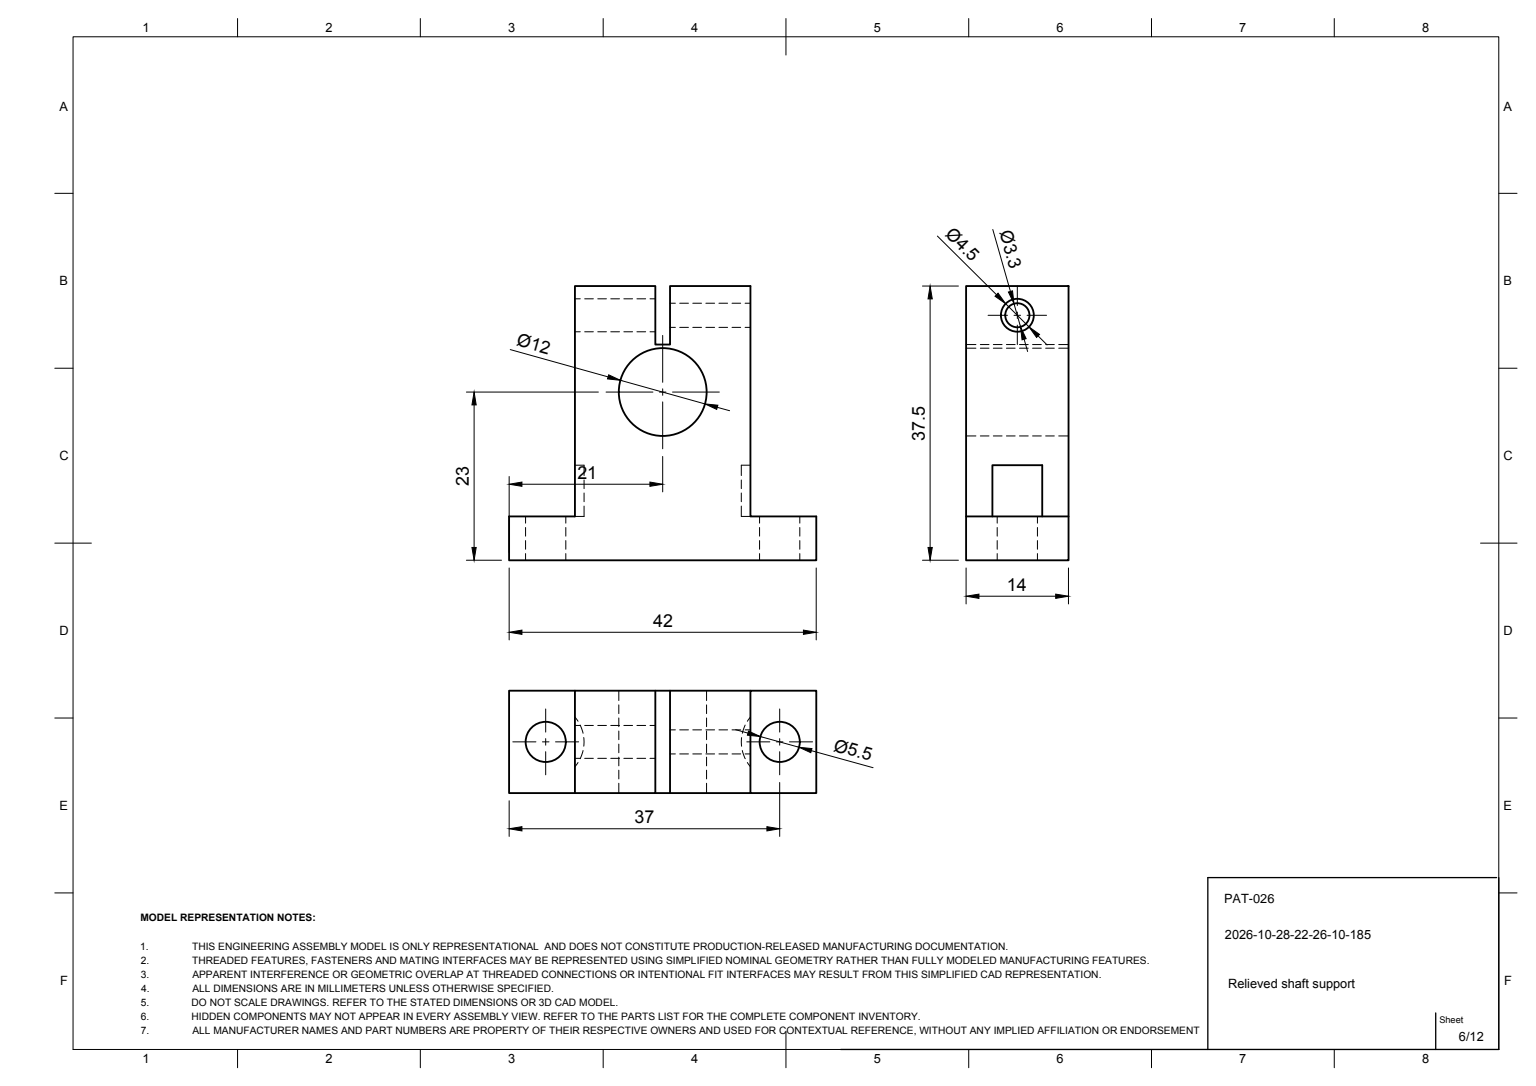
ISO-10303-21;
HEADER;
/* Generated by software containing ST-Developer
 * from STEP Tools, Inc. (www.steptools.com) 
 */

FILE_DESCRIPTION(
/* description */ ('PAT-026'),
/* implementation_level */ '2;1');

FILE_NAME(
/* name */ 'Relieved shaft support.step',
/* time_stamp */ '2026-10-28T22:25:58-07:00',
/* author */ (''),
/* organization */ (''),
/* preprocessor_version */ 'ST-DEVELOPER v20.2',
/* originating_system */ 'Autodesk Translation Framework v15.17.0.0',
/* authorisation */ '');

FILE_SCHEMA (('AUTOMOTIVE_DESIGN { 1 0 10303 214 3 1 1 }'));
ENDSEC;

DATA;
#10=MECHANICAL_DESIGN_GEOMETRIC_PRESENTATION_REPRESENTATION('',(#144),#12343);
#122=SHAPE_REPRESENTATION_RELATIONSHIP('SRR','None',#12399,#133);
#133=ADVANCED_BREP_SHAPE_REPRESENTATION('',(#155),#12334);
#144=STYLED_ITEM('',(#12533),#155);
#155=MANIFOLD_SOLID_BREP('Body1',#7350);
#169=FACE_BOUND('',#985,.T.);
#170=FACE_BOUND('',#987,.T.);
#171=FACE_BOUND('',#989,.T.);
#172=FACE_BOUND('',#996,.T.);
#173=FACE_BOUND('',#999,.T.);
#174=FACE_BOUND('',#1000,.T.);
#175=FACE_BOUND('',#1003,.T.);
#176=FACE_BOUND('',#1006,.T.);
#177=FACE_BOUND('',#1009,.T.);
#178=FACE_BOUND('',#1012,.T.);
#204=PLANE('',#7515);
#205=PLANE('',#7522);
#206=PLANE('',#7523);
#207=PLANE('',#7525);
#208=PLANE('',#7527);
#209=PLANE('',#7541);
#210=PLANE('',#7542);
#211=PLANE('',#7543);
#212=PLANE('',#7544);
#213=PLANE('',#7545);
#214=PLANE('',#7546);
#215=PLANE('',#7547);
#216=PLANE('',#7548);
#217=PLANE('',#7549);
#218=PLANE('',#7550);
#219=PLANE('',#7551);
#569=FACE_OUTER_BOUND('',#980,.T.);
#570=FACE_OUTER_BOUND('',#981,.T.);
#571=FACE_OUTER_BOUND('',#982,.T.);
#572=FACE_OUTER_BOUND('',#983,.T.);
#573=FACE_OUTER_BOUND('',#984,.T.);
#574=FACE_OUTER_BOUND('',#986,.T.);
#575=FACE_OUTER_BOUND('',#988,.T.);
#576=FACE_OUTER_BOUND('',#990,.T.);
#577=FACE_OUTER_BOUND('',#991,.T.);
#578=FACE_OUTER_BOUND('',#992,.T.);
#579=FACE_OUTER_BOUND('',#993,.T.);
#580=FACE_OUTER_BOUND('',#994,.T.);
#581=FACE_OUTER_BOUND('',#995,.T.);
#582=FACE_OUTER_BOUND('',#997,.T.);
#583=FACE_OUTER_BOUND('',#998,.T.);
#584=FACE_OUTER_BOUND('',#1001,.T.);
#585=FACE_OUTER_BOUND('',#1002,.T.);
#586=FACE_OUTER_BOUND('',#1004,.T.);
#587=FACE_OUTER_BOUND('',#1005,.T.);
#588=FACE_OUTER_BOUND('',#1007,.T.);
#589=FACE_OUTER_BOUND('',#1008,.T.);
#590=FACE_OUTER_BOUND('',#1010,.T.);
#591=FACE_OUTER_BOUND('',#1011,.T.);
#980=EDGE_LOOP('',(#4959,#4960));
#981=EDGE_LOOP('',(#4961,#4962,#4963,#4964));
#982=EDGE_LOOP('',(#4965,#4966,#4967,#4968));
#983=EDGE_LOOP('',(#4969,#4970));
#984=EDGE_LOOP('',(#4971,#4972,#4973,#4974,#4975,#4976));
#985=EDGE_LOOP('',(#4977));
#986=EDGE_LOOP('',(#4978,#4979,#4980,#4981,#4982,#4983,#4984,#4985));
#987=EDGE_LOOP('',(#4986));
#988=EDGE_LOOP('',(#4987,#4988,#4989,#4990,#4991,#4992));
#989=EDGE_LOOP('',(#4993));
#990=EDGE_LOOP('',(#4994,#4995,#4996,#4997));
#991=EDGE_LOOP('',(#4998,#4999,#5000,#5001));
#992=EDGE_LOOP('',(#5002,#5003,#5004,#5005));
#993=EDGE_LOOP('',(#5006,#5007,#5008,#5009));
#994=EDGE_LOOP('',(#5010,#5011,#5012,#5013));
#995=EDGE_LOOP('',(#5014,#5015,#5016,#5017,#5018,#5019,#5020,#5021,#5022,
#5023,#5024,#5025));
#996=EDGE_LOOP('',(#5026));
#997=EDGE_LOOP('',(#5027,#5028,#5029,#5030));
#998=EDGE_LOOP('',(#5031,#5032,#5033,#5034));
#999=EDGE_LOOP('',(#5035));
#1000=EDGE_LOOP('',(#5036));
#1001=EDGE_LOOP('',(#5037,#5038,#5039,#5040));
#1002=EDGE_LOOP('',(#5041,#5042,#5043,#5044,#5045,#5046,#5047,#5048));
#1003=EDGE_LOOP('',(#5049));
#1004=EDGE_LOOP('',(#5050,#5051,#5052,#5053));
#1005=EDGE_LOOP('',(#5054,#5055,#5056,#5057));
#1006=EDGE_LOOP('',(#5058));
#1007=EDGE_LOOP('',(#5059,#5060,#5061,#5062));
#1008=EDGE_LOOP('',(#5063,#5064,#5065,#5066));
#1009=EDGE_LOOP('',(#5067));
#1010=EDGE_LOOP('',(#5068,#5069,#5070,#5071));
#1011=EDGE_LOOP('',(#5072,#5073,#5074,#5075,#5076,#5077,#5078,#5079,#5080,
#5081,#5082,#5083));
#1012=EDGE_LOOP('',(#5084));
#1410=LINE('',#10114,#2282);
#1411=LINE('',#10118,#2283);
#1412=LINE('',#10121,#2284);
#1413=LINE('',#10125,#2285);
#1414=LINE('',#10129,#2286);
#1415=LINE('',#10132,#2287);
#1416=LINE('',#10135,#2288);
#1417=LINE('',#10137,#2289);
#1418=LINE('',#10139,#2290);
#1419=LINE('',#10141,#2291);
#1420=LINE('',#10142,#2292);
#1421=LINE('',#10147,#2293);
#1422=LINE('',#10149,#2294);
#1423=LINE('',#10150,#2295);
#1424=LINE('',#10156,#2296);
#1425=LINE('',#10158,#2297);
#1426=LINE('',#10159,#2298);
#1427=LINE('',#10161,#2299);
#1428=LINE('',#10162,#2300);
#1429=LINE('',#10169,#2301);
#1430=LINE('',#10173,#2302);
#1431=LINE('',#10178,#2303);
#1432=LINE('',#10182,#2304);
#1433=LINE('',#10187,#2305);
#1434=LINE('',#10191,#2306);
#1435=LINE('',#10193,#2307);
#1436=LINE('',#10194,#2308);
#1437=LINE('',#10196,#2309);
#1438=LINE('',#10198,#2310);
#1439=LINE('',#10200,#2311);
#1440=LINE('',#10202,#2312);
#1441=LINE('',#10204,#2313);
#1442=LINE('',#10205,#2314);
#1443=LINE('',#10208,#2315);
#1444=LINE('',#10209,#2316);
#1445=LINE('',#10212,#2317);
#1446=LINE('',#10213,#2318);
#1447=LINE('',#10215,#2319);
#1448=LINE('',#10218,#2320);
#1449=LINE('',#10219,#2321);
#1450=LINE('',#10222,#2322);
#1451=LINE('',#10223,#2323);
#1452=LINE('',#10226,#2324);
#1453=LINE('',#10227,#2325);
#1454=LINE('',#10230,#2326);
#1455=LINE('',#10231,#2327);
#1456=LINE('',#10234,#2328);
#1457=LINE('',#10235,#2329);
#1458=LINE('',#10237,#2330);
#2282=VECTOR('',#8130,1.);
#2283=VECTOR('',#8135,1.);
#2284=VECTOR('',#8138,1.);
#2285=VECTOR('',#8141,1.);
#2286=VECTOR('',#8144,1.);
#2287=VECTOR('',#8149,1.);
#2288=VECTOR('',#8152,1.);
#2289=VECTOR('',#8153,1.);
#2290=VECTOR('',#8154,1.);
#2291=VECTOR('',#8155,1.);
#2292=VECTOR('',#8156,1.);
#2293=VECTOR('',#8161,1.);
#2294=VECTOR('',#8162,1.);
#2295=VECTOR('',#8163,1.);
#2296=VECTOR('',#8168,1.);
#2297=VECTOR('',#8169,1.);
#2298=VECTOR('',#8170,1.);
#2299=VECTOR('',#8171,1.);
#2300=VECTOR('',#8172,1.);
#2301=VECTOR('',#8179,0.225);
#2302=VECTOR('',#8184,0.165);
#2303=VECTOR('',#8191,0.275);
#2304=VECTOR('',#8196,0.275);
#2305=VECTOR('',#8201,0.6);
#2306=VECTOR('',#8206,1.);
#2307=VECTOR('',#8207,1.);
#2308=VECTOR('',#8208,1.);
#2309=VECTOR('',#8209,1.);
#2310=VECTOR('',#8210,1.);
#2311=VECTOR('',#8211,1.);
#2312=VECTOR('',#8212,1.);
#2313=VECTOR('',#8213,1.);
#2314=VECTOR('',#8214,1.);
#2315=VECTOR('',#8217,1.);
#2316=VECTOR('',#8218,1.);
#2317=VECTOR('',#8221,1.);
#2318=VECTOR('',#8222,1.);
#2319=VECTOR('',#8225,1.);
#2320=VECTOR('',#8228,1.);
#2321=VECTOR('',#8229,1.);
#2322=VECTOR('',#8232,1.);
#2323=VECTOR('',#8233,1.);
#2324=VECTOR('',#8236,1.);
#2325=VECTOR('',#8237,1.);
#2326=VECTOR('',#8240,1.);
#2327=VECTOR('',#8241,1.);
#2328=VECTOR('',#8244,1.);
#2329=VECTOR('',#8245,1.);
#2330=VECTOR('',#8248,1.);
#3148=CIRCLE('',#7516,0.525);
#3149=CIRCLE('',#7518,0.525);
#3150=CIRCLE('',#7520,0.525);
#3151=CIRCLE('',#7521,0.525);
#3152=CIRCLE('',#7524,0.275);
#3153=CIRCLE('',#7526,0.165);
#3154=CIRCLE('',#7528,0.275);
#3155=CIRCLE('',#7530,0.225);
#3156=CIRCLE('',#7531,0.225);
#3157=CIRCLE('',#7533,0.165);
#3158=CIRCLE('',#7535,0.275);
#3159=CIRCLE('',#7537,0.275);
#3160=CIRCLE('',#7539,0.6);
#3161=CIRCLE('',#7540,0.6);
#3281=VERTEX_POINT('',#10112);
#3282=VERTEX_POINT('',#10113);
#3283=VERTEX_POINT('',#10117);
#3284=VERTEX_POINT('',#10119);
#3285=VERTEX_POINT('',#10123);
#3286=VERTEX_POINT('',#10124);
#3287=VERTEX_POINT('',#10126);
#3288=VERTEX_POINT('',#10128);
#3289=VERTEX_POINT('',#10134);
#3290=VERTEX_POINT('',#10136);
#3291=VERTEX_POINT('',#10138);
#3292=VERTEX_POINT('',#10140);
#3293=VERTEX_POINT('',#10143);
#3294=VERTEX_POINT('',#10146);
#3295=VERTEX_POINT('',#10148);
#3296=VERTEX_POINT('',#10151);
#3297=VERTEX_POINT('',#10154);
#3298=VERTEX_POINT('',#10155);
#3299=VERTEX_POINT('',#10157);
#3300=VERTEX_POINT('',#10160);
#3301=VERTEX_POINT('',#10163);
#3302=VERTEX_POINT('',#10166);
#3303=VERTEX_POINT('',#10168);
#3304=VERTEX_POINT('',#10172);
#3305=VERTEX_POINT('',#10176);
#3306=VERTEX_POINT('',#10180);
#3307=VERTEX_POINT('',#10184);
#3308=VERTEX_POINT('',#10186);
#3309=VERTEX_POINT('',#10190);
#3310=VERTEX_POINT('',#10192);
#3311=VERTEX_POINT('',#10195);
#3312=VERTEX_POINT('',#10197);
#3313=VERTEX_POINT('',#10199);
#3314=VERTEX_POINT('',#10201);
#3315=VERTEX_POINT('',#10203);
#3316=VERTEX_POINT('',#10207);
#3317=VERTEX_POINT('',#10211);
#3318=VERTEX_POINT('',#10217);
#3319=VERTEX_POINT('',#10221);
#3320=VERTEX_POINT('',#10225);
#3321=VERTEX_POINT('',#10229);
#3322=VERTEX_POINT('',#10233);
#3923=EDGE_CURVE('',#3281,#3282,#1410,.T.);
#3924=EDGE_CURVE('',#3282,#3281,#3148,.T.);
#3925=EDGE_CURVE('',#3283,#3281,#1411,.T.);
#3926=EDGE_CURVE('',#3284,#3283,#3149,.T.);
#3927=EDGE_CURVE('',#3282,#3284,#1412,.T.);
#3928=EDGE_CURVE('',#3285,#3286,#1413,.T.);
#3929=EDGE_CURVE('',#3285,#3287,#3150,.T.);
#3930=EDGE_CURVE('',#3288,#3287,#1414,.T.);
#3931=EDGE_CURVE('',#3286,#3288,#3151,.T.);
#3932=EDGE_CURVE('',#3287,#3285,#1415,.T.);
#3933=EDGE_CURVE('',#3283,#3289,#1416,.T.);
#3934=EDGE_CURVE('',#3290,#3289,#1417,.T.);
#3935=EDGE_CURVE('',#3290,#3291,#1418,.T.);
#3936=EDGE_CURVE('',#3292,#3291,#1419,.T.);
#3937=EDGE_CURVE('',#3292,#3284,#1420,.T.);
#3938=EDGE_CURVE('',#3293,#3293,#3152,.T.);
#3939=EDGE_CURVE('',#3294,#3292,#1421,.T.);
#3940=EDGE_CURVE('',#3294,#3295,#1422,.T.);
#3941=EDGE_CURVE('',#3289,#3295,#1423,.T.);
#3942=EDGE_CURVE('',#3296,#3296,#3153,.T.);
#3943=EDGE_CURVE('',#3297,#3298,#1424,.T.);
#3944=EDGE_CURVE('',#3299,#3298,#1425,.T.);
#3945=EDGE_CURVE('',#3286,#3299,#1426,.T.);
#3946=EDGE_CURVE('',#3300,#3288,#1427,.T.);
#3947=EDGE_CURVE('',#3297,#3300,#1428,.T.);
#3948=EDGE_CURVE('',#3301,#3301,#3154,.T.);
#3949=EDGE_CURVE('',#3302,#3302,#3155,.T.);
#3950=EDGE_CURVE('',#3302,#3303,#1429,.T.);
#3951=EDGE_CURVE('',#3303,#3303,#3156,.T.);
#3952=EDGE_CURVE('',#3296,#3304,#1430,.T.);
#3953=EDGE_CURVE('',#3304,#3304,#3157,.T.);
#3954=EDGE_CURVE('',#3305,#3305,#3158,.T.);
#3955=EDGE_CURVE('',#3305,#3293,#1431,.T.);
#3956=EDGE_CURVE('',#3306,#3306,#3159,.T.);
#3957=EDGE_CURVE('',#3306,#3301,#1432,.T.);
#3958=EDGE_CURVE('',#3307,#3307,#3160,.T.);
#3959=EDGE_CURVE('',#3307,#3308,#1433,.T.);
#3960=EDGE_CURVE('',#3308,#3308,#3161,.T.);
#3961=EDGE_CURVE('',#3291,#3309,#1434,.T.);
#3962=EDGE_CURVE('',#3309,#3310,#1435,.T.);
#3963=EDGE_CURVE('',#3310,#3297,#1436,.T.);
#3964=EDGE_CURVE('',#3300,#3311,#1437,.T.);
#3965=EDGE_CURVE('',#3311,#3312,#1438,.T.);
#3966=EDGE_CURVE('',#3312,#3313,#1439,.T.);
#3967=EDGE_CURVE('',#3313,#3314,#1440,.T.);
#3968=EDGE_CURVE('',#3314,#3315,#1441,.T.);
#3969=EDGE_CURVE('',#3315,#3294,#1442,.T.);
#3970=EDGE_CURVE('',#3316,#3290,#1443,.T.);
#3971=EDGE_CURVE('',#3309,#3316,#1444,.T.);
#3972=EDGE_CURVE('',#3317,#3316,#1445,.T.);
#3973=EDGE_CURVE('',#3310,#3317,#1446,.T.);
#3974=EDGE_CURVE('',#3298,#3317,#1447,.T.);
#3975=EDGE_CURVE('',#3318,#3299,#1448,.T.);
#3976=EDGE_CURVE('',#3311,#3318,#1449,.T.);
#3977=EDGE_CURVE('',#3319,#3318,#1450,.T.);
#3978=EDGE_CURVE('',#3312,#3319,#1451,.T.);
#3979=EDGE_CURVE('',#3320,#3319,#1452,.T.);
#3980=EDGE_CURVE('',#3313,#3320,#1453,.T.);
#3981=EDGE_CURVE('',#3321,#3320,#1454,.T.);
#3982=EDGE_CURVE('',#3314,#3321,#1455,.T.);
#3983=EDGE_CURVE('',#3322,#3321,#1456,.T.);
#3984=EDGE_CURVE('',#3315,#3322,#1457,.T.);
#3985=EDGE_CURVE('',#3295,#3322,#1458,.T.);
#4959=ORIENTED_EDGE('',*,*,#3923,.F.);
#4960=ORIENTED_EDGE('',*,*,#3924,.F.);
#4961=ORIENTED_EDGE('',*,*,#3925,.F.);
#4962=ORIENTED_EDGE('',*,*,#3926,.F.);
#4963=ORIENTED_EDGE('',*,*,#3927,.F.);
#4964=ORIENTED_EDGE('',*,*,#3924,.T.);
#4965=ORIENTED_EDGE('',*,*,#3928,.F.);
#4966=ORIENTED_EDGE('',*,*,#3929,.T.);
#4967=ORIENTED_EDGE('',*,*,#3930,.F.);
#4968=ORIENTED_EDGE('',*,*,#3931,.F.);
#4969=ORIENTED_EDGE('',*,*,#3932,.F.);
#4970=ORIENTED_EDGE('',*,*,#3929,.F.);
#4971=ORIENTED_EDGE('',*,*,#3933,.T.);
#4972=ORIENTED_EDGE('',*,*,#3934,.F.);
#4973=ORIENTED_EDGE('',*,*,#3935,.T.);
#4974=ORIENTED_EDGE('',*,*,#3936,.F.);
#4975=ORIENTED_EDGE('',*,*,#3937,.T.);
#4976=ORIENTED_EDGE('',*,*,#3926,.T.);
#4977=ORIENTED_EDGE('',*,*,#3938,.T.);
#4978=ORIENTED_EDGE('',*,*,#3925,.T.);
#4979=ORIENTED_EDGE('',*,*,#3923,.T.);
#4980=ORIENTED_EDGE('',*,*,#3927,.T.);
#4981=ORIENTED_EDGE('',*,*,#3937,.F.);
#4982=ORIENTED_EDGE('',*,*,#3939,.F.);
#4983=ORIENTED_EDGE('',*,*,#3940,.T.);
#4984=ORIENTED_EDGE('',*,*,#3941,.F.);
#4985=ORIENTED_EDGE('',*,*,#3933,.F.);
#4986=ORIENTED_EDGE('',*,*,#3942,.T.);
#4987=ORIENTED_EDGE('',*,*,#3943,.T.);
#4988=ORIENTED_EDGE('',*,*,#3944,.F.);
#4989=ORIENTED_EDGE('',*,*,#3945,.F.);
#4990=ORIENTED_EDGE('',*,*,#3931,.T.);
#4991=ORIENTED_EDGE('',*,*,#3946,.F.);
#4992=ORIENTED_EDGE('',*,*,#3947,.F.);
#4993=ORIENTED_EDGE('',*,*,#3948,.T.);
#4994=ORIENTED_EDGE('',*,*,#3949,.F.);
#4995=ORIENTED_EDGE('',*,*,#3950,.T.);
#4996=ORIENTED_EDGE('',*,*,#3951,.F.);
#4997=ORIENTED_EDGE('',*,*,#3950,.F.);
#4998=ORIENTED_EDGE('',*,*,#3942,.F.);
#4999=ORIENTED_EDGE('',*,*,#3952,.T.);
#5000=ORIENTED_EDGE('',*,*,#3953,.F.);
#5001=ORIENTED_EDGE('',*,*,#3952,.F.);
#5002=ORIENTED_EDGE('',*,*,#3954,.F.);
#5003=ORIENTED_EDGE('',*,*,#3955,.T.);
#5004=ORIENTED_EDGE('',*,*,#3938,.F.);
#5005=ORIENTED_EDGE('',*,*,#3955,.F.);
#5006=ORIENTED_EDGE('',*,*,#3956,.F.);
#5007=ORIENTED_EDGE('',*,*,#3957,.T.);
#5008=ORIENTED_EDGE('',*,*,#3948,.F.);
#5009=ORIENTED_EDGE('',*,*,#3957,.F.);
#5010=ORIENTED_EDGE('',*,*,#3958,.F.);
#5011=ORIENTED_EDGE('',*,*,#3959,.T.);
#5012=ORIENTED_EDGE('',*,*,#3960,.F.);
#5013=ORIENTED_EDGE('',*,*,#3959,.F.);
#5014=ORIENTED_EDGE('',*,*,#3936,.T.);
#5015=ORIENTED_EDGE('',*,*,#3961,.T.);
#5016=ORIENTED_EDGE('',*,*,#3962,.T.);
#5017=ORIENTED_EDGE('',*,*,#3963,.T.);
#5018=ORIENTED_EDGE('',*,*,#3947,.T.);
#5019=ORIENTED_EDGE('',*,*,#3964,.T.);
#5020=ORIENTED_EDGE('',*,*,#3965,.T.);
#5021=ORIENTED_EDGE('',*,*,#3966,.T.);
#5022=ORIENTED_EDGE('',*,*,#3967,.T.);
#5023=ORIENTED_EDGE('',*,*,#3968,.T.);
#5024=ORIENTED_EDGE('',*,*,#3969,.T.);
#5025=ORIENTED_EDGE('',*,*,#3939,.T.);
#5026=ORIENTED_EDGE('',*,*,#3958,.T.);
#5027=ORIENTED_EDGE('',*,*,#3935,.F.);
#5028=ORIENTED_EDGE('',*,*,#3970,.F.);
#5029=ORIENTED_EDGE('',*,*,#3971,.F.);
#5030=ORIENTED_EDGE('',*,*,#3961,.F.);
#5031=ORIENTED_EDGE('',*,*,#3971,.T.);
#5032=ORIENTED_EDGE('',*,*,#3972,.F.);
#5033=ORIENTED_EDGE('',*,*,#3973,.F.);
#5034=ORIENTED_EDGE('',*,*,#3962,.F.);
#5035=ORIENTED_EDGE('',*,*,#3954,.T.);
#5036=ORIENTED_EDGE('',*,*,#3956,.T.);
#5037=ORIENTED_EDGE('',*,*,#3973,.T.);
#5038=ORIENTED_EDGE('',*,*,#3974,.F.);
#5039=ORIENTED_EDGE('',*,*,#3943,.F.);
#5040=ORIENTED_EDGE('',*,*,#3963,.F.);
#5041=ORIENTED_EDGE('',*,*,#3928,.T.);
#5042=ORIENTED_EDGE('',*,*,#3945,.T.);
#5043=ORIENTED_EDGE('',*,*,#3975,.F.);
#5044=ORIENTED_EDGE('',*,*,#3976,.F.);
#5045=ORIENTED_EDGE('',*,*,#3964,.F.);
#5046=ORIENTED_EDGE('',*,*,#3946,.T.);
#5047=ORIENTED_EDGE('',*,*,#3930,.T.);
#5048=ORIENTED_EDGE('',*,*,#3932,.T.);
#5049=ORIENTED_EDGE('',*,*,#3951,.T.);
#5050=ORIENTED_EDGE('',*,*,#3976,.T.);
#5051=ORIENTED_EDGE('',*,*,#3977,.F.);
#5052=ORIENTED_EDGE('',*,*,#3978,.F.);
#5053=ORIENTED_EDGE('',*,*,#3965,.F.);
#5054=ORIENTED_EDGE('',*,*,#3978,.T.);
#5055=ORIENTED_EDGE('',*,*,#3979,.F.);
#5056=ORIENTED_EDGE('',*,*,#3980,.F.);
#5057=ORIENTED_EDGE('',*,*,#3966,.F.);
#5058=ORIENTED_EDGE('',*,*,#3949,.T.);
#5059=ORIENTED_EDGE('',*,*,#3980,.T.);
#5060=ORIENTED_EDGE('',*,*,#3981,.F.);
#5061=ORIENTED_EDGE('',*,*,#3982,.F.);
#5062=ORIENTED_EDGE('',*,*,#3967,.F.);
#5063=ORIENTED_EDGE('',*,*,#3982,.T.);
#5064=ORIENTED_EDGE('',*,*,#3983,.F.);
#5065=ORIENTED_EDGE('',*,*,#3984,.F.);
#5066=ORIENTED_EDGE('',*,*,#3968,.F.);
#5067=ORIENTED_EDGE('',*,*,#3953,.T.);
#5068=ORIENTED_EDGE('',*,*,#3984,.T.);
#5069=ORIENTED_EDGE('',*,*,#3985,.F.);
#5070=ORIENTED_EDGE('',*,*,#3940,.F.);
#5071=ORIENTED_EDGE('',*,*,#3969,.F.);
#5072=ORIENTED_EDGE('',*,*,#3934,.T.);
#5073=ORIENTED_EDGE('',*,*,#3941,.T.);
#5074=ORIENTED_EDGE('',*,*,#3985,.T.);
#5075=ORIENTED_EDGE('',*,*,#3983,.T.);
#5076=ORIENTED_EDGE('',*,*,#3981,.T.);
#5077=ORIENTED_EDGE('',*,*,#3979,.T.);
#5078=ORIENTED_EDGE('',*,*,#3977,.T.);
#5079=ORIENTED_EDGE('',*,*,#3975,.T.);
#5080=ORIENTED_EDGE('',*,*,#3944,.T.);
#5081=ORIENTED_EDGE('',*,*,#3974,.T.);
#5082=ORIENTED_EDGE('',*,*,#3972,.T.);
#5083=ORIENTED_EDGE('',*,*,#3970,.T.);
#5084=ORIENTED_EDGE('',*,*,#3960,.T.);
#6917=CYLINDRICAL_SURFACE('',#7517,0.525);
#6918=CYLINDRICAL_SURFACE('',#7519,0.525);
#6919=CYLINDRICAL_SURFACE('',#7529,0.225);
#6920=CYLINDRICAL_SURFACE('',#7532,0.165);
#6921=CYLINDRICAL_SURFACE('',#7534,0.275);
#6922=CYLINDRICAL_SURFACE('',#7536,0.275);
#6923=CYLINDRICAL_SURFACE('',#7538,0.6);
#6960=ADVANCED_FACE('',(#569),#204,.F.);
#6961=ADVANCED_FACE('',(#570),#6917,.F.);
#6962=ADVANCED_FACE('',(#571),#6918,.F.);
#6963=ADVANCED_FACE('',(#572),#205,.F.);
#6964=ADVANCED_FACE('',(#573,#169),#206,.T.);
#6965=ADVANCED_FACE('',(#574,#170),#207,.T.);
#6966=ADVANCED_FACE('',(#575,#171),#208,.T.);
#6967=ADVANCED_FACE('',(#576),#6919,.F.);
#6968=ADVANCED_FACE('',(#577),#6920,.F.);
#6969=ADVANCED_FACE('',(#578),#6921,.F.);
#6970=ADVANCED_FACE('',(#579),#6922,.F.);
#6971=ADVANCED_FACE('',(#580),#6923,.F.);
#6972=ADVANCED_FACE('',(#581,#172),#209,.T.);
#6973=ADVANCED_FACE('',(#582),#210,.T.);
#6974=ADVANCED_FACE('',(#583,#173,#174),#211,.T.);
#6975=ADVANCED_FACE('',(#584),#212,.T.);
#6976=ADVANCED_FACE('',(#585,#175),#213,.T.);
#6977=ADVANCED_FACE('',(#586),#214,.T.);
#6978=ADVANCED_FACE('',(#587,#176),#215,.T.);
#6979=ADVANCED_FACE('',(#588),#216,.T.);
#6980=ADVANCED_FACE('',(#589,#177),#217,.T.);
#6981=ADVANCED_FACE('',(#590),#218,.T.);
#6982=ADVANCED_FACE('',(#591,#178),#219,.T.);
#7350=CLOSED_SHELL('',(#6960,#6961,#6962,#6963,#6964,#6965,#6966,#6967,
#6968,#6969,#6970,#6971,#6972,#6973,#6974,#6975,#6976,#6977,#6978,#6979,
#6980,#6981,#6982));
#7514=AXIS2_PLACEMENT_3D('',#10110,#8126,#8127);
#7515=AXIS2_PLACEMENT_3D('',#10111,#8128,#8129);
#7516=AXIS2_PLACEMENT_3D('',#10115,#8131,#8132);
#7517=AXIS2_PLACEMENT_3D('',#10116,#8133,#8134);
#7518=AXIS2_PLACEMENT_3D('',#10120,#8136,#8137);
#7519=AXIS2_PLACEMENT_3D('',#10122,#8139,#8140);
#7520=AXIS2_PLACEMENT_3D('',#10127,#8142,#8143);
#7521=AXIS2_PLACEMENT_3D('',#10130,#8145,#8146);
#7522=AXIS2_PLACEMENT_3D('',#10131,#8147,#8148);
#7523=AXIS2_PLACEMENT_3D('',#10133,#8150,#8151);
#7524=AXIS2_PLACEMENT_3D('',#10144,#8157,#8158);
#7525=AXIS2_PLACEMENT_3D('',#10145,#8159,#8160);
#7526=AXIS2_PLACEMENT_3D('',#10152,#8164,#8165);
#7527=AXIS2_PLACEMENT_3D('',#10153,#8166,#8167);
#7528=AXIS2_PLACEMENT_3D('',#10164,#8173,#8174);
#7529=AXIS2_PLACEMENT_3D('',#10165,#8175,#8176);
#7530=AXIS2_PLACEMENT_3D('',#10167,#8177,#8178);
#7531=AXIS2_PLACEMENT_3D('',#10170,#8180,#8181);
#7532=AXIS2_PLACEMENT_3D('',#10171,#8182,#8183);
#7533=AXIS2_PLACEMENT_3D('',#10174,#8185,#8186);
#7534=AXIS2_PLACEMENT_3D('',#10175,#8187,#8188);
#7535=AXIS2_PLACEMENT_3D('',#10177,#8189,#8190);
#7536=AXIS2_PLACEMENT_3D('',#10179,#8192,#8193);
#7537=AXIS2_PLACEMENT_3D('',#10181,#8194,#8195);
#7538=AXIS2_PLACEMENT_3D('',#10183,#8197,#8198);
#7539=AXIS2_PLACEMENT_3D('',#10185,#8199,#8200);
#7540=AXIS2_PLACEMENT_3D('',#10188,#8202,#8203);
#7541=AXIS2_PLACEMENT_3D('',#10189,#8204,#8205);
#7542=AXIS2_PLACEMENT_3D('',#10206,#8215,#8216);
#7543=AXIS2_PLACEMENT_3D('',#10210,#8219,#8220);
#7544=AXIS2_PLACEMENT_3D('',#10214,#8223,#8224);
#7545=AXIS2_PLACEMENT_3D('',#10216,#8226,#8227);
#7546=AXIS2_PLACEMENT_3D('',#10220,#8230,#8231);
#7547=AXIS2_PLACEMENT_3D('',#10224,#8234,#8235);
#7548=AXIS2_PLACEMENT_3D('',#10228,#8238,#8239);
#7549=AXIS2_PLACEMENT_3D('',#10232,#8242,#8243);
#7550=AXIS2_PLACEMENT_3D('',#10236,#8246,#8247);
#7551=AXIS2_PLACEMENT_3D('',#10238,#8249,#8250);
#8126=DIRECTION('axis',(0.,0.,1.));
#8127=DIRECTION('refdir',(1.,0.,0.));
#8128=DIRECTION('center_axis',(0.,0.,1.));
#8129=DIRECTION('ref_axis',(1.,0.,0.));
#8130=DIRECTION('',(0.,-1.,0.));
#8131=DIRECTION('center_axis',(0.,0.,1.));
#8132=DIRECTION('ref_axis',(1.,0.,0.));
#8133=DIRECTION('center_axis',(0.,0.,1.));
#8134=DIRECTION('ref_axis',(1.,0.,0.));
#8135=DIRECTION('',(0.,0.,1.));
#8136=DIRECTION('center_axis',(0.,0.,1.));
#8137=DIRECTION('ref_axis',(1.,0.,0.));
#8138=DIRECTION('',(0.,0.,-1.));
#8139=DIRECTION('center_axis',(0.,0.,1.));
#8140=DIRECTION('ref_axis',(-1.,1.22464679914735E-16,0.));
#8141=DIRECTION('',(0.,0.,-1.));
#8142=DIRECTION('center_axis',(0.,0.,1.));
#8143=DIRECTION('ref_axis',(1.,0.,0.));
#8144=DIRECTION('',(0.,0.,1.));
#8145=DIRECTION('center_axis',(0.,0.,1.));
#8146=DIRECTION('ref_axis',(1.,0.,0.));
#8147=DIRECTION('center_axis',(0.,0.,1.));
#8148=DIRECTION('ref_axis',(1.,0.,0.));
#8149=DIRECTION('',(0.,1.,0.));
#8150=DIRECTION('center_axis',(0.,0.,1.));
#8151=DIRECTION('ref_axis',(1.,0.,0.));
#8152=DIRECTION('',(0.,1.,0.));
#8153=DIRECTION('',(1.,0.,0.));
#8154=DIRECTION('',(0.,-1.,0.));
#8155=DIRECTION('',(-1.,0.,0.));
#8156=DIRECTION('',(0.,1.,0.));
#8157=DIRECTION('center_axis',(0.,0.,-1.));
#8158=DIRECTION('ref_axis',(1.,0.,0.));
#8159=DIRECTION('center_axis',(-1.,0.,0.));
#8160=DIRECTION('ref_axis',(0.,0.,1.));
#8161=DIRECTION('',(0.,0.,-1.));
#8162=DIRECTION('',(0.,1.,0.));
#8163=DIRECTION('',(0.,0.,1.));
#8164=DIRECTION('center_axis',(1.,0.,0.));
#8165=DIRECTION('ref_axis',(0.,0.,-1.));
#8166=DIRECTION('center_axis',(0.,0.,1.));
#8167=DIRECTION('ref_axis',(1.,0.,0.));
#8168=DIRECTION('',(0.,1.,0.));
#8169=DIRECTION('',(1.,0.,0.));
#8170=DIRECTION('',(0.,1.,0.));
#8171=DIRECTION('',(0.,1.,0.));
#8172=DIRECTION('',(-1.,0.,0.));
#8173=DIRECTION('center_axis',(0.,0.,-1.));
#8174=DIRECTION('ref_axis',(1.,0.,0.));
#8175=DIRECTION('center_axis',(1.,0.,0.));
#8176=DIRECTION('ref_axis',(0.,0.,-1.));
#8177=DIRECTION('center_axis',(1.,0.,0.));
#8178=DIRECTION('ref_axis',(0.,0.,-1.));
#8179=DIRECTION('',(1.,0.,0.));
#8180=DIRECTION('center_axis',(-1.,0.,0.));
#8181=DIRECTION('ref_axis',(0.,0.,-1.));
#8182=DIRECTION('center_axis',(1.,0.,0.));
#8183=DIRECTION('ref_axis',(0.,0.,-1.));
#8184=DIRECTION('',(1.,0.,0.));
#8185=DIRECTION('center_axis',(-1.,0.,0.));
#8186=DIRECTION('ref_axis',(0.,0.,-1.));
#8187=DIRECTION('center_axis',(0.,0.,1.));
#8188=DIRECTION('ref_axis',(1.,0.,0.));
#8189=DIRECTION('center_axis',(0.,0.,1.));
#8190=DIRECTION('ref_axis',(1.,0.,0.));
#8191=DIRECTION('',(0.,0.,1.));
#8192=DIRECTION('center_axis',(0.,0.,1.));
#8193=DIRECTION('ref_axis',(1.,0.,0.));
#8194=DIRECTION('center_axis',(0.,0.,1.));
#8195=DIRECTION('ref_axis',(1.,0.,0.));
#8196=DIRECTION('',(0.,0.,1.));
#8197=DIRECTION('center_axis',(0.,1.,0.));
#8198=DIRECTION('ref_axis',(1.,0.,0.));
#8199=DIRECTION('center_axis',(0.,1.,0.));
#8200=DIRECTION('ref_axis',(1.,0.,0.));
#8201=DIRECTION('',(0.,1.,0.));
#8202=DIRECTION('center_axis',(0.,-1.,0.));
#8203=DIRECTION('ref_axis',(1.,0.,0.));
#8204=DIRECTION('center_axis',(0.,-1.,0.));
#8205=DIRECTION('ref_axis',(0.,0.,-1.));
#8206=DIRECTION('',(0.,0.,-1.));
#8207=DIRECTION('',(1.,0.,0.));
#8208=DIRECTION('',(0.,0.,1.));
#8209=DIRECTION('',(0.,0.,1.));
#8210=DIRECTION('',(-1.,0.,0.));
#8211=DIRECTION('',(0.,0.,-1.));
#8212=DIRECTION('',(-1.,0.,0.));
#8213=DIRECTION('',(0.,0.,1.));
#8214=DIRECTION('',(-1.,0.,0.));
#8215=DIRECTION('center_axis',(-1.,0.,0.));
#8216=DIRECTION('ref_axis',(0.,0.,1.));
#8217=DIRECTION('',(0.,0.,1.));
#8218=DIRECTION('',(0.,1.,0.));
#8219=DIRECTION('center_axis',(0.,0.,-1.));
#8220=DIRECTION('ref_axis',(-1.,0.,0.));
#8221=DIRECTION('',(-1.,0.,0.));
#8222=DIRECTION('',(0.,1.,0.));
#8223=DIRECTION('center_axis',(1.,0.,0.));
#8224=DIRECTION('ref_axis',(0.,0.,-1.));
#8225=DIRECTION('',(0.,0.,-1.));
#8226=DIRECTION('center_axis',(1.,0.,0.));
#8227=DIRECTION('ref_axis',(0.,0.,-1.));
#8228=DIRECTION('',(0.,0.,-1.));
#8229=DIRECTION('',(0.,1.,0.));
#8230=DIRECTION('center_axis',(0.,0.,1.));
#8231=DIRECTION('ref_axis',(1.,0.,0.));
#8232=DIRECTION('',(1.,0.,0.));
#8233=DIRECTION('',(0.,1.,0.));
#8234=DIRECTION('center_axis',(-1.,0.,0.));
#8235=DIRECTION('ref_axis',(0.,0.,1.));
#8236=DIRECTION('',(0.,0.,1.));
#8237=DIRECTION('',(0.,1.,0.));
#8238=DIRECTION('center_axis',(0.,0.,1.));
#8239=DIRECTION('ref_axis',(1.,0.,0.));
#8240=DIRECTION('',(1.,0.,0.));
#8241=DIRECTION('',(0.,1.,0.));
#8242=DIRECTION('center_axis',(1.,0.,0.));
#8243=DIRECTION('ref_axis',(0.,0.,-1.));
#8244=DIRECTION('',(0.,0.,-1.));
#8245=DIRECTION('',(0.,1.,0.));
#8246=DIRECTION('center_axis',(0.,0.,1.));
#8247=DIRECTION('ref_axis',(1.,0.,0.));
#8248=DIRECTION('',(1.,0.,0.));
#8249=DIRECTION('center_axis',(0.,1.,0.));
#8250=DIRECTION('ref_axis',(0.,0.,1.));
#10110=CARTESIAN_POINT('',(0.,0.,0.));
#10111=CARTESIAN_POINT('Origin',(-1.6,0.,1.3));
#10112=CARTESIAN_POINT('',(-1.2,0.340036762718386,1.3));
#10113=CARTESIAN_POINT('',(-1.2,-0.340036762718386,1.3));
#10114=CARTESIAN_POINT('',(-1.2,0.,1.3));
#10115=CARTESIAN_POINT('Origin',(-1.6,0.,1.3));
#10116=CARTESIAN_POINT('Origin',(-1.6,0.,0.6));
#10117=CARTESIAN_POINT('',(-1.2,0.340036762718386,0.6));
#10118=CARTESIAN_POINT('',(-1.2,0.340036762718386,0.6));
#10119=CARTESIAN_POINT('',(-1.2,-0.340036762718386,0.6));
#10120=CARTESIAN_POINT('Origin',(-1.6,0.,0.6));
#10121=CARTESIAN_POINT('',(-1.2,-0.340036762718386,0.6));
#10122=CARTESIAN_POINT('Origin',(1.6,0.,0.6));
#10123=CARTESIAN_POINT('',(1.2,0.340036762718386,1.3));
#10124=CARTESIAN_POINT('',(1.2,0.340036762718386,0.6));
#10125=CARTESIAN_POINT('',(1.2,0.340036762718386,0.6));
#10126=CARTESIAN_POINT('',(1.2,-0.340036762718386,1.3));
#10127=CARTESIAN_POINT('Origin',(1.6,0.,1.3));
#10128=CARTESIAN_POINT('',(1.2,-0.340036762718386,0.6));
#10129=CARTESIAN_POINT('',(1.2,-0.340036762718386,0.6));
#10130=CARTESIAN_POINT('Origin',(1.6,0.,0.6));
#10131=CARTESIAN_POINT('Origin',(1.6,0.,1.3));
#10132=CARTESIAN_POINT('',(1.2,0.,1.3));
#10133=CARTESIAN_POINT('Origin',(-2.1,0.,0.6));
#10134=CARTESIAN_POINT('',(-1.2,0.7,0.6));
#10135=CARTESIAN_POINT('',(-1.2,0.,0.6));
#10136=CARTESIAN_POINT('',(-2.1,0.7,0.6));
#10137=CARTESIAN_POINT('',(-1.2,0.7,0.6));
#10138=CARTESIAN_POINT('',(-2.1,-0.7,0.6));
#10139=CARTESIAN_POINT('',(-2.1,0.,0.6));
#10140=CARTESIAN_POINT('',(-1.2,-0.7,0.6));
#10141=CARTESIAN_POINT('',(-1.2,-0.7,0.6));
#10142=CARTESIAN_POINT('',(-1.2,0.,0.6));
#10143=CARTESIAN_POINT('',(-1.875,3.36777869765522E-17,0.6));
#10144=CARTESIAN_POINT('Origin',(-1.6,0.,0.6));
#10145=CARTESIAN_POINT('Origin',(-1.2,0.,0.6));
#10146=CARTESIAN_POINT('',(-1.2,-0.7,3.75));
#10147=CARTESIAN_POINT('',(-1.2,-0.7,3.75));
#10148=CARTESIAN_POINT('',(-1.2,0.7,3.75));
#10149=CARTESIAN_POINT('',(-1.2,0.,3.75));
#10150=CARTESIAN_POINT('',(-1.2,0.7,3.75));
#10151=CARTESIAN_POINT('',(-1.2,-2.02066721859313E-17,3.515));
#10152=CARTESIAN_POINT('Origin',(-1.2,0.,3.35));
#10153=CARTESIAN_POINT('Origin',(1.2,0.,0.6));
#10154=CARTESIAN_POINT('',(2.1,-0.7,0.6));
#10155=CARTESIAN_POINT('',(2.1,0.7,0.6));
#10156=CARTESIAN_POINT('',(2.1,0.,0.6));
#10157=CARTESIAN_POINT('',(1.2,0.7,0.6));
#10158=CARTESIAN_POINT('',(2.1,0.7,0.6));
#10159=CARTESIAN_POINT('',(1.2,0.,0.6));
#10160=CARTESIAN_POINT('',(1.2,-0.7,0.6));
#10161=CARTESIAN_POINT('',(1.2,0.,0.6));
#10162=CARTESIAN_POINT('',(2.1,-0.7,0.6));
#10163=CARTESIAN_POINT('',(1.325,3.36777869765522E-17,0.6));
#10164=CARTESIAN_POINT('Origin',(1.6,0.,0.6));
#10165=CARTESIAN_POINT('Origin',(0.1,0.,3.35));
#10166=CARTESIAN_POINT('',(0.1,-2.75545529808155E-17,3.575));
#10167=CARTESIAN_POINT('Origin',(0.1,0.,3.35));
#10168=CARTESIAN_POINT('',(1.2,2.75545529808155E-17,3.575));
#10169=CARTESIAN_POINT('',(0.1,-2.75545529808155E-17,3.575));
#10170=CARTESIAN_POINT('Origin',(1.2,0.,3.35));
#10171=CARTESIAN_POINT('Origin',(0.,0.,3.35));
#10172=CARTESIAN_POINT('',(-0.1,2.02066721859313E-17,3.515));
#10173=CARTESIAN_POINT('',(0.,-2.02066721859313E-17,3.515));
#10174=CARTESIAN_POINT('Origin',(-0.1,0.,3.35));
#10175=CARTESIAN_POINT('Origin',(-1.6,0.,-0.05));
#10176=CARTESIAN_POINT('',(-1.875,-3.36777869765522E-17,0.));
#10177=CARTESIAN_POINT('Origin',(-1.6,0.,0.));
#10178=CARTESIAN_POINT('',(-1.875,-3.36777869765522E-17,-0.05));
#10179=CARTESIAN_POINT('Origin',(1.6,0.,-0.05));
#10180=CARTESIAN_POINT('',(1.325,-3.36777869765522E-17,0.));
#10181=CARTESIAN_POINT('Origin',(1.6,0.,0.));
#10182=CARTESIAN_POINT('',(1.325,-3.36777869765522E-17,-0.05));
#10183=CARTESIAN_POINT('Origin',(0.,0.,2.3));
#10184=CARTESIAN_POINT('',(-0.6,-0.7,2.3));
#10185=CARTESIAN_POINT('Origin',(0.,-0.7,2.3));
#10186=CARTESIAN_POINT('',(-0.6,0.7,2.3));
#10187=CARTESIAN_POINT('',(-0.6,0.,2.3));
#10188=CARTESIAN_POINT('Origin',(0.,0.7,2.3));
#10189=CARTESIAN_POINT('Origin',(0.,-0.7,1.875));
#10190=CARTESIAN_POINT('',(-2.1,-0.7,0.));
#10191=CARTESIAN_POINT('',(-2.1,-0.7,0.6));
#10192=CARTESIAN_POINT('',(2.1,-0.7,0.));
#10193=CARTESIAN_POINT('',(-2.1,-0.7,0.));
#10194=CARTESIAN_POINT('',(2.1,-0.7,0.));
#10195=CARTESIAN_POINT('',(1.2,-0.7,3.75));
#10196=CARTESIAN_POINT('',(1.2,-0.7,0.6));
#10197=CARTESIAN_POINT('',(0.1,-0.7,3.75));
#10198=CARTESIAN_POINT('',(1.2,-0.7,3.75));
#10199=CARTESIAN_POINT('',(0.1,-0.7,2.95));
#10200=CARTESIAN_POINT('',(0.1,-0.7,3.75));
#10201=CARTESIAN_POINT('',(-0.1,-0.7,2.95));
#10202=CARTESIAN_POINT('',(0.1,-0.7,2.95));
#10203=CARTESIAN_POINT('',(-0.1,-0.7,3.75));
#10204=CARTESIAN_POINT('',(-0.1,-0.7,2.95));
#10205=CARTESIAN_POINT('',(-0.1,-0.7,3.75));
#10206=CARTESIAN_POINT('Origin',(-2.1,0.,0.));
#10207=CARTESIAN_POINT('',(-2.1,0.7,0.));
#10208=CARTESIAN_POINT('',(-2.1,0.7,0.6));
#10209=CARTESIAN_POINT('',(-2.1,0.,0.));
#10210=CARTESIAN_POINT('Origin',(2.1,0.,0.));
#10211=CARTESIAN_POINT('',(2.1,0.7,0.));
#10212=CARTESIAN_POINT('',(-2.1,0.7,0.));
#10213=CARTESIAN_POINT('',(2.1,0.,0.));
#10214=CARTESIAN_POINT('Origin',(2.1,0.,0.6));
#10215=CARTESIAN_POINT('',(2.1,0.7,0.));
#10216=CARTESIAN_POINT('Origin',(1.2,0.,3.75));
#10217=CARTESIAN_POINT('',(1.2,0.7,3.75));
#10218=CARTESIAN_POINT('',(1.2,0.7,0.6));
#10219=CARTESIAN_POINT('',(1.2,0.,3.75));
#10220=CARTESIAN_POINT('Origin',(0.1,0.,3.75));
#10221=CARTESIAN_POINT('',(0.1,0.7,3.75));
#10222=CARTESIAN_POINT('',(1.2,0.7,3.75));
#10223=CARTESIAN_POINT('',(0.1,0.,3.75));
#10224=CARTESIAN_POINT('Origin',(0.1,0.,2.95));
#10225=CARTESIAN_POINT('',(0.1,0.7,2.95));
#10226=CARTESIAN_POINT('',(0.1,0.7,3.75));
#10227=CARTESIAN_POINT('',(0.1,0.,2.95));
#10228=CARTESIAN_POINT('Origin',(-0.1,0.,2.95));
#10229=CARTESIAN_POINT('',(-0.1,0.7,2.95));
#10230=CARTESIAN_POINT('',(0.1,0.7,2.95));
#10231=CARTESIAN_POINT('',(-0.1,0.,2.95));
#10232=CARTESIAN_POINT('Origin',(-0.1,0.,3.75));
#10233=CARTESIAN_POINT('',(-0.1,0.7,3.75));
#10234=CARTESIAN_POINT('',(-0.1,0.7,2.95));
#10235=CARTESIAN_POINT('',(-0.1,0.,3.75));
#10236=CARTESIAN_POINT('Origin',(-1.2,0.,3.75));
#10237=CARTESIAN_POINT('',(-0.1,0.7,3.75));
#10238=CARTESIAN_POINT('Origin',(0.,0.7,1.875));
#12320=UNCERTAINTY_MEASURE_WITH_UNIT(LENGTH_MEASURE(0.001),#12344,
'DISTANCE_ACCURACY_VALUE',
'Maximum model space distance between geometric entities at asserted c
onnectivities');
#12329=UNCERTAINTY_MEASURE_WITH_UNIT(LENGTH_MEASURE(0.001),#12344,
'DISTANCE_ACCURACY_VALUE',
'Maximum model space distance between geometric entities at asserted c
onnectivities');
#12334=(
GEOMETRIC_REPRESENTATION_CONTEXT(3)
GLOBAL_UNCERTAINTY_ASSIGNED_CONTEXT((#12320))
GLOBAL_UNIT_ASSIGNED_CONTEXT((#12344,#12346,#12347))
REPRESENTATION_CONTEXT('','3D')
);
#12343=(
GEOMETRIC_REPRESENTATION_CONTEXT(3)
GLOBAL_UNCERTAINTY_ASSIGNED_CONTEXT((#12329))
GLOBAL_UNIT_ASSIGNED_CONTEXT((#12344,#12346,#12347))
REPRESENTATION_CONTEXT('','3D')
);
#12344=(
LENGTH_UNIT()
NAMED_UNIT(*)
SI_UNIT(.CENTI.,.METRE.)
);
#12346=(
NAMED_UNIT(*)
PLANE_ANGLE_UNIT()
SI_UNIT($,.RADIAN.)
);
#12347=(
NAMED_UNIT(*)
SI_UNIT($,.STERADIAN.)
SOLID_ANGLE_UNIT()
);
#12352=SHAPE_DEFINITION_REPRESENTATION(#12365,#12399);
#12365=PRODUCT_DEFINITION_SHAPE('',$,#12413);
#12399=SHAPE_REPRESENTATION('',(#7514),#12334);
#12408=PRODUCT_DEFINITION_CONTEXT('part definition',#12449,'design');
#12413=PRODUCT_DEFINITION('Relieved shaft support',
'Relieved shaft support',#12426,#12408);
#12426=PRODUCT_DEFINITION_FORMATION('',$,#12455);
#12449=APPLICATION_CONTEXT(
'Core Data for Automotive Mechanical Design Process');
#12450=PRODUCT_CONTEXT('part definition',#12449,'mechanical');
#12455=PRODUCT('Relieved shaft support','Relieved shaft support',
'Relieved shaft support',(#12450));
#12527=COLOUR_RGB('Grey',0.48,0.52,0.57);
#12528=FILL_AREA_STYLE_COLOUR('',#12527);
#12529=FILL_AREA_STYLE('',(#12528));
#12530=SURFACE_STYLE_FILL_AREA(#12529);
#12531=SURFACE_SIDE_STYLE('',(#12530));
#12532=SURFACE_STYLE_USAGE(.BOTH.,#12531);
#12533=PRESENTATION_STYLE_ASSIGNMENT((#12532));
ENDSEC;
END-ISO-10303-21;
